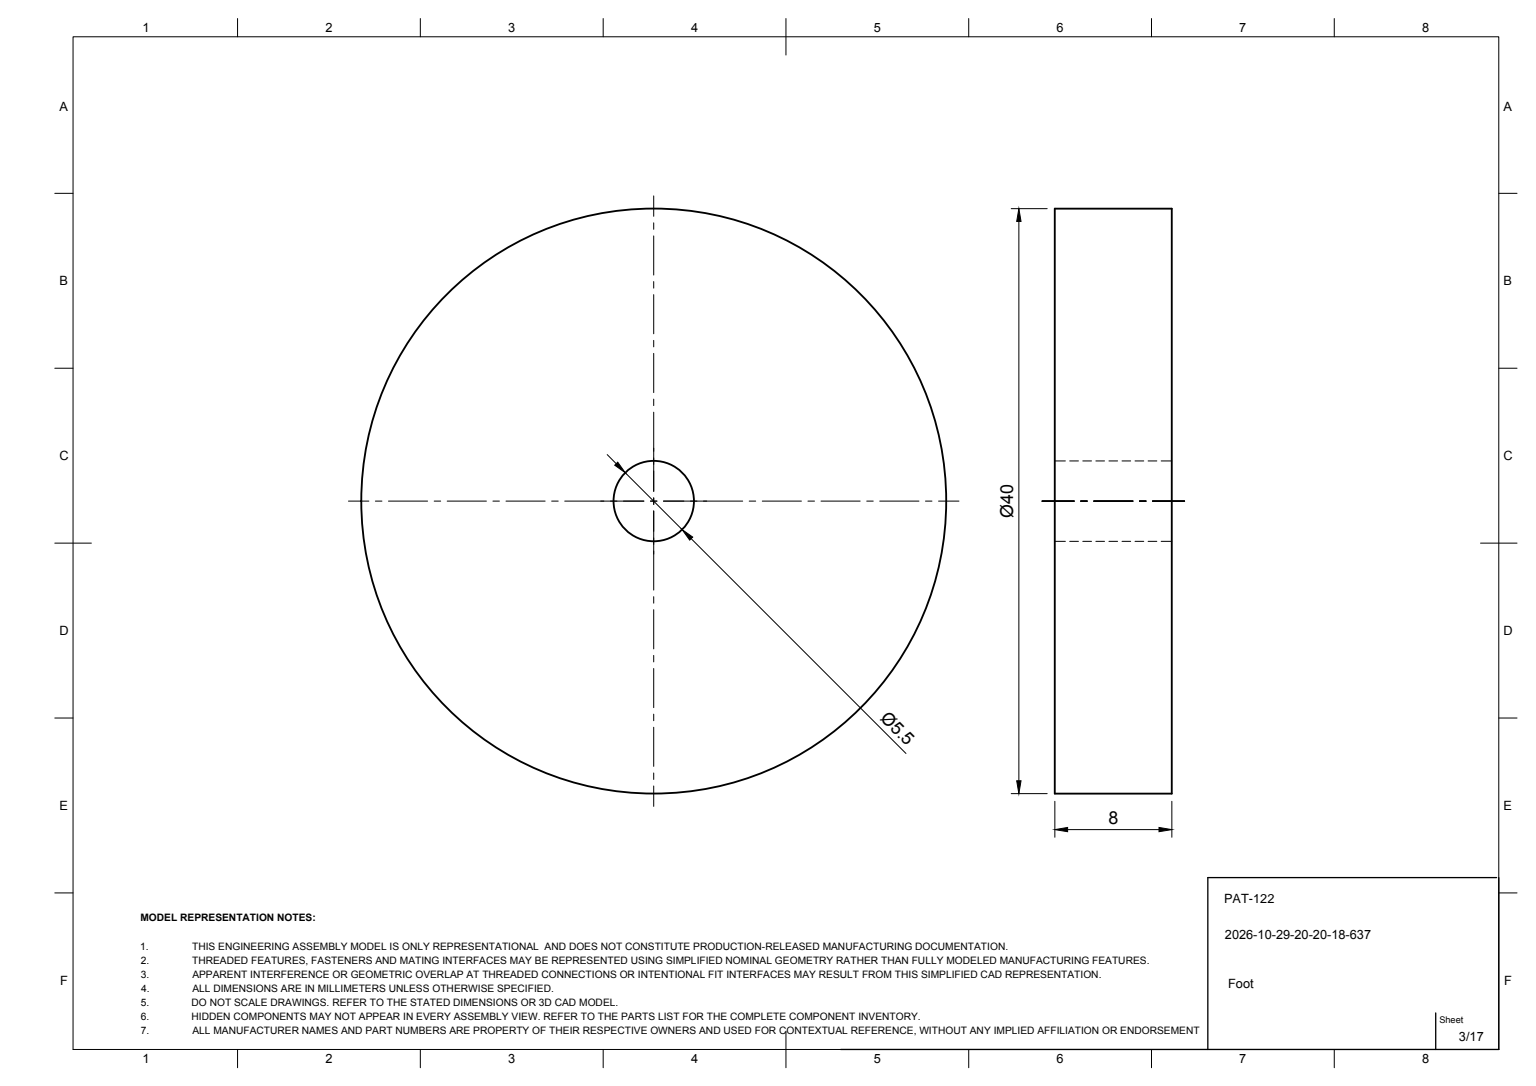
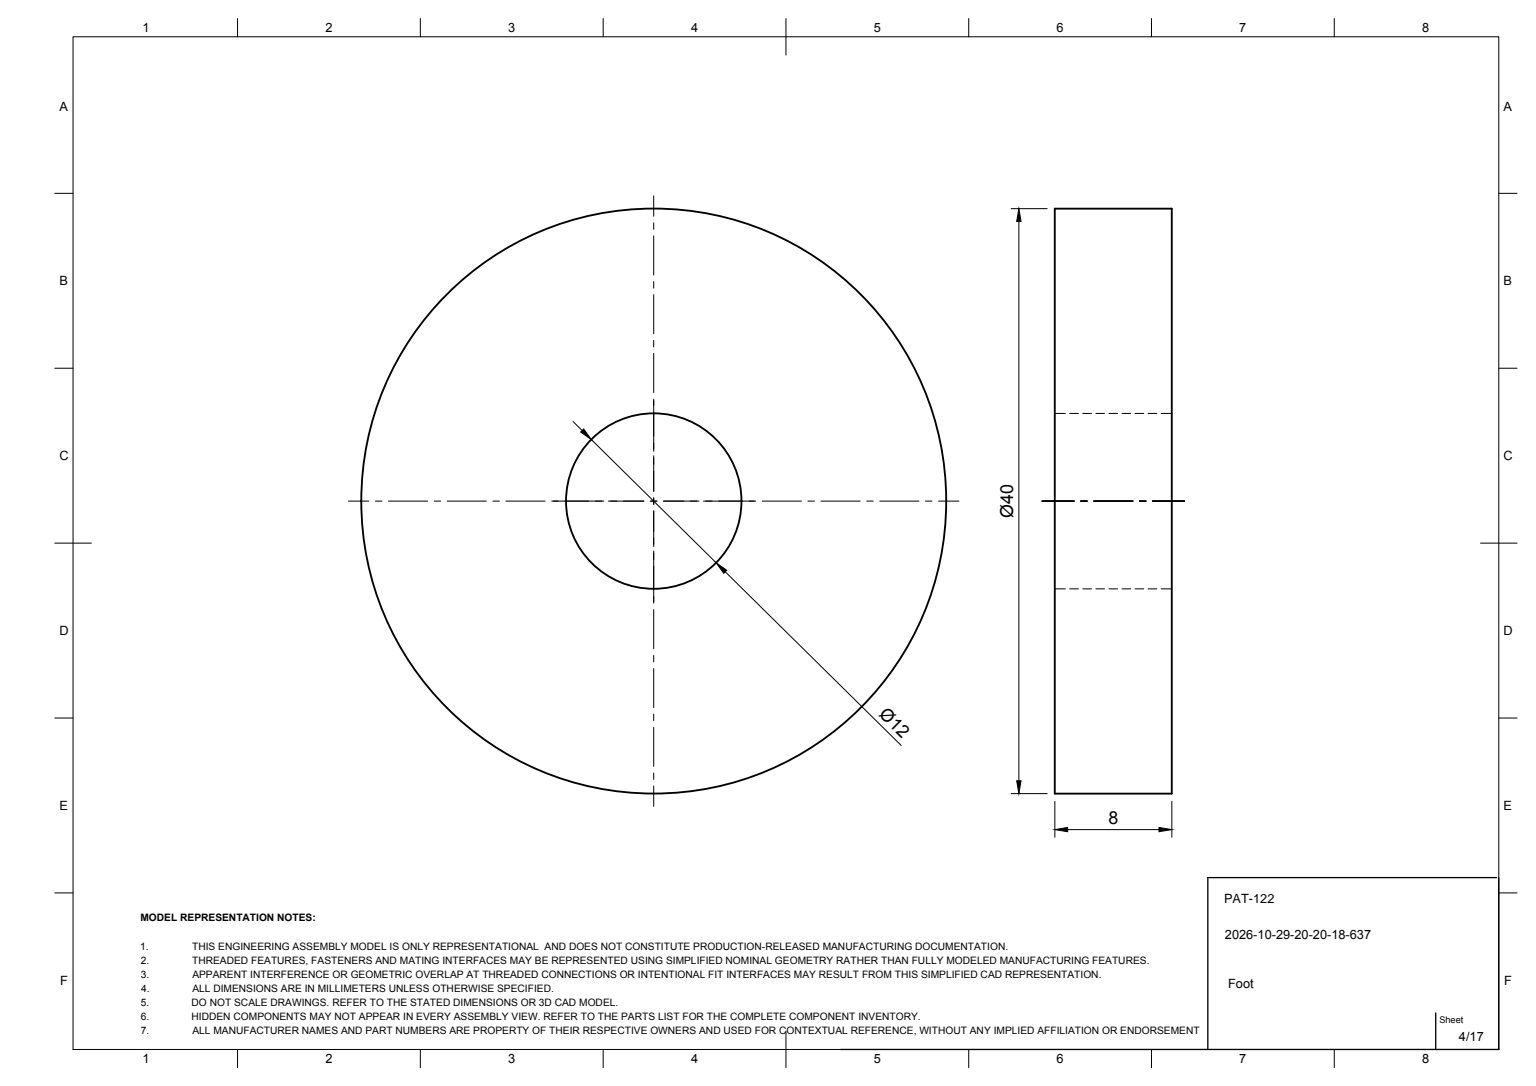
ISO-10303-21;
HEADER;
/* Generated by software containing ST-Developer
 * from STEP Tools, Inc. (www.steptools.com) 
 */

FILE_DESCRIPTION(
/* description */ ('PAT-122'),
/* implementation_level */ '2;1');

FILE_NAME(
/* name */ 'Foot.step',
/* time_stamp */ '2026-10-29T20:20:12-07:00',
/* author */ (''),
/* organization */ (''),
/* preprocessor_version */ 'ST-DEVELOPER v20.2',
/* originating_system */ 'Autodesk Translation Framework v15.17.0.0',
/* authorisation */ '');

FILE_SCHEMA (('AUTOMOTIVE_DESIGN { 1 0 10303 214 3 1 1 }'));
ENDSEC;

DATA;
#10=MECHANICAL_DESIGN_GEOMETRIC_PRESENTATION_REPRESENTATION('',(#491),#10019);
#447=SHAPE_REPRESENTATION_RELATIONSHIP('SRR','None',#10168,#469);
#469=ADVANCED_BREP_SHAPE_REPRESENTATION('',(#513),#9997);
#491=STYLED_ITEM('',(#10362),#513);
#513=MANIFOLD_SOLID_BREP('Body1',#5613);
#531=FACE_BOUND('',#1120,.T.);
#532=FACE_BOUND('',#1122,.T.);
#609=PLANE('',#5890);
#610=PLANE('',#5891);
#825=FACE_OUTER_BOUND('',#1117,.T.);
#826=FACE_OUTER_BOUND('',#1118,.T.);
#827=FACE_OUTER_BOUND('',#1119,.T.);
#828=FACE_OUTER_BOUND('',#1121,.T.);
#1117=EDGE_LOOP('',(#3865,#3866,#3867,#3868));
#1118=EDGE_LOOP('',(#3869,#3870,#3871,#3872));
#1119=EDGE_LOOP('',(#3873));
#1120=EDGE_LOOP('',(#3874));
#1121=EDGE_LOOP('',(#3875));
#1122=EDGE_LOOP('',(#3876));
#1487=LINE('',#8064,#2031);
#1488=LINE('',#8070,#2032);
#2031=VECTOR('',#6434,0.274999999999999);
#2032=VECTOR('',#6441,2.);
#2575=CIRCLE('',#5885,0.274999999999999);
#2576=CIRCLE('',#5886,0.274999999999999);
#2577=CIRCLE('',#5888,2.);
#2578=CIRCLE('',#5889,2.);
#2705=VERTEX_POINT('',#8061);
#2706=VERTEX_POINT('',#8063);
#2707=VERTEX_POINT('',#8067);
#2708=VERTEX_POINT('',#8069);
#3167=EDGE_CURVE('',#2705,#2705,#2575,.T.);
#3168=EDGE_CURVE('',#2705,#2706,#1487,.T.);
#3169=EDGE_CURVE('',#2706,#2706,#2576,.T.);
#3170=EDGE_CURVE('',#2707,#2707,#2577,.T.);
#3171=EDGE_CURVE('',#2707,#2708,#1488,.T.);
#3172=EDGE_CURVE('',#2708,#2708,#2578,.T.);
#3865=ORIENTED_EDGE('',*,*,#3167,.F.);
#3866=ORIENTED_EDGE('',*,*,#3168,.T.);
#3867=ORIENTED_EDGE('',*,*,#3169,.T.);
#3868=ORIENTED_EDGE('',*,*,#3168,.F.);
#3869=ORIENTED_EDGE('',*,*,#3170,.F.);
#3870=ORIENTED_EDGE('',*,*,#3171,.T.);
#3871=ORIENTED_EDGE('',*,*,#3172,.T.);
#3872=ORIENTED_EDGE('',*,*,#3171,.F.);
#3873=ORIENTED_EDGE('',*,*,#3170,.T.);
#3874=ORIENTED_EDGE('',*,*,#3167,.T.);
#3875=ORIENTED_EDGE('',*,*,#3172,.F.);
#3876=ORIENTED_EDGE('',*,*,#3169,.F.);
#5261=CYLINDRICAL_SURFACE('',#5884,0.274999999999999);
#5262=CYLINDRICAL_SURFACE('',#5887,2.);
#5321=ADVANCED_FACE('',(#825),#5261,.F.);
#5322=ADVANCED_FACE('',(#826),#5262,.T.);
#5323=ADVANCED_FACE('',(#827,#531),#609,.T.);
#5324=ADVANCED_FACE('',(#828,#532),#610,.F.);
#5613=CLOSED_SHELL('',(#5321,#5322,#5323,#5324));
#5883=AXIS2_PLACEMENT_3D('',#8059,#6428,#6429);
#5884=AXIS2_PLACEMENT_3D('',#8060,#6430,#6431);
#5885=AXIS2_PLACEMENT_3D('',#8062,#6432,#6433);
#5886=AXIS2_PLACEMENT_3D('',#8065,#6435,#6436);
#5887=AXIS2_PLACEMENT_3D('',#8066,#6437,#6438);
#5888=AXIS2_PLACEMENT_3D('',#8068,#6439,#6440);
#5889=AXIS2_PLACEMENT_3D('',#8071,#6442,#6443);
#5890=AXIS2_PLACEMENT_3D('',#8072,#6444,#6445);
#5891=AXIS2_PLACEMENT_3D('',#8073,#6446,#6447);
#6428=DIRECTION('axis',(0.,0.,1.));
#6429=DIRECTION('refdir',(1.,0.,0.));
#6430=DIRECTION('center_axis',(0.,0.,1.));
#6431=DIRECTION('ref_axis',(1.,0.,0.));
#6432=DIRECTION('center_axis',(0.,0.,-1.));
#6433=DIRECTION('ref_axis',(1.,0.,0.));
#6434=DIRECTION('',(0.,0.,-1.));
#6435=DIRECTION('center_axis',(0.,0.,-1.));
#6436=DIRECTION('ref_axis',(1.,0.,0.));
#6437=DIRECTION('center_axis',(0.,0.,1.));
#6438=DIRECTION('ref_axis',(1.,0.,0.));
#6439=DIRECTION('center_axis',(0.,0.,1.));
#6440=DIRECTION('ref_axis',(1.,0.,0.));
#6441=DIRECTION('',(0.,0.,-1.));
#6442=DIRECTION('center_axis',(0.,0.,1.));
#6443=DIRECTION('ref_axis',(1.,0.,0.));
#6444=DIRECTION('center_axis',(0.,0.,1.));
#6445=DIRECTION('ref_axis',(1.,0.,0.));
#6446=DIRECTION('center_axis',(0.,0.,1.));
#6447=DIRECTION('ref_axis',(1.,0.,0.));
#8059=CARTESIAN_POINT('',(0.,0.,0.));
#8060=CARTESIAN_POINT('Origin',(-19.,-19.,-0.8));
#8061=CARTESIAN_POINT('',(-19.275,-19.,0.));
#8062=CARTESIAN_POINT('Origin',(-19.,-19.,0.));
#8063=CARTESIAN_POINT('',(-19.275,-19.,-0.8));
#8064=CARTESIAN_POINT('',(-19.275,-19.,-0.8));
#8065=CARTESIAN_POINT('Origin',(-19.,-19.,-0.8));
#8066=CARTESIAN_POINT('Origin',(-19.,-19.,-0.8));
#8067=CARTESIAN_POINT('',(-21.,-19.,0.));
#8068=CARTESIAN_POINT('Origin',(-19.,-19.,0.));
#8069=CARTESIAN_POINT('',(-21.,-19.,-0.8));
#8070=CARTESIAN_POINT('',(-21.,-19.,-0.8));
#8071=CARTESIAN_POINT('Origin',(-19.,-19.,-0.8));
#8072=CARTESIAN_POINT('Origin',(-19.,-19.,0.));
#8073=CARTESIAN_POINT('Origin',(-19.,-19.,-0.8));
#9973=UNCERTAINTY_MEASURE_WITH_UNIT(LENGTH_MEASURE(0.001),#10020,
'DISTANCE_ACCURACY_VALUE',
'Maximum model space distance between geometric entities at asserted c
onnectivities');
#9995=UNCERTAINTY_MEASURE_WITH_UNIT(LENGTH_MEASURE(0.001),#10020,
'DISTANCE_ACCURACY_VALUE',
'Maximum model space distance between geometric entities at asserted c
onnectivities');
#9997=(
GEOMETRIC_REPRESENTATION_CONTEXT(3)
GLOBAL_UNCERTAINTY_ASSIGNED_CONTEXT((#9973))
GLOBAL_UNIT_ASSIGNED_CONTEXT((#10020,#10022,#10023))
REPRESENTATION_CONTEXT('','3D')
);
#10019=(
GEOMETRIC_REPRESENTATION_CONTEXT(3)
GLOBAL_UNCERTAINTY_ASSIGNED_CONTEXT((#9995))
GLOBAL_UNIT_ASSIGNED_CONTEXT((#10020,#10022,#10023))
REPRESENTATION_CONTEXT('','3D')
);
#10020=(
LENGTH_UNIT()
NAMED_UNIT(*)
SI_UNIT(.CENTI.,.METRE.)
);
#10022=(
NAMED_UNIT(*)
PLANE_ANGLE_UNIT()
SI_UNIT($,.RADIAN.)
);
#10023=(
NAMED_UNIT(*)
SI_UNIT($,.STERADIAN.)
SOLID_ANGLE_UNIT()
);
#10025=SHAPE_DEFINITION_REPRESENTATION(#10048,#10168);
#10048=PRODUCT_DEFINITION_SHAPE('',$,#10192);
#10168=SHAPE_REPRESENTATION('',(#5883),#9997);
#10190=PRODUCT_DEFINITION_CONTEXT('part definition',#10261,'design');
#10192=PRODUCT_DEFINITION('Foot','Foot',#10215,#10190);
#10215=PRODUCT_DEFINITION_FORMATION('',$,#10264);
#10261=APPLICATION_CONTEXT(
'Core Data for Automotive Mechanical Design Process');
#10262=PRODUCT_CONTEXT('part definition',#10261,'mechanical');
#10264=PRODUCT('Foot','Foot','Foot',(#10262));
#10356=COLOUR_RGB('Off White',0.89,0.88,0.83);
#10357=FILL_AREA_STYLE_COLOUR('',#10356);
#10358=FILL_AREA_STYLE('',(#10357));
#10359=SURFACE_STYLE_FILL_AREA(#10358);
#10360=SURFACE_SIDE_STYLE('',(#10359));
#10361=SURFACE_STYLE_USAGE(.BOTH.,#10360);
#10362=PRESENTATION_STYLE_ASSIGNMENT((#10361));
ENDSEC;
END-ISO-10303-21;
